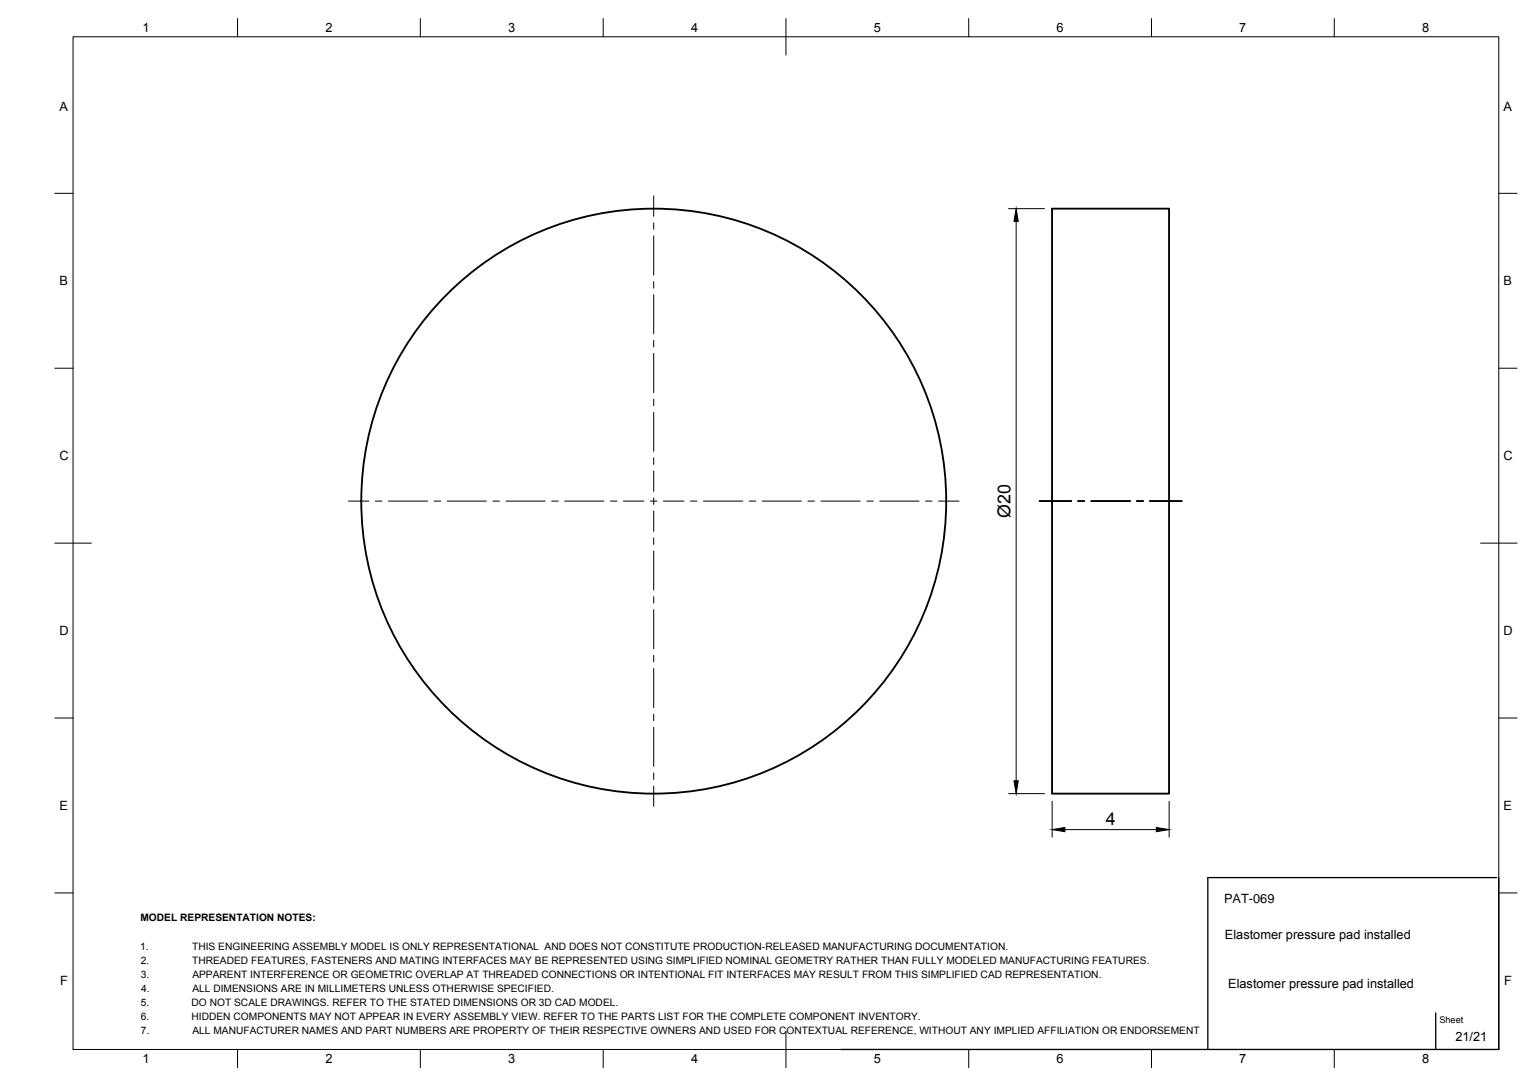
ISO-10303-21;
HEADER;
/* Generated by software containing ST-Developer
 * from STEP Tools, Inc. (www.steptools.com) 
 */

FILE_DESCRIPTION(
/* description */ ('Located fixture plate with toggle clamp'),
/* implementation_level */ '2;1');

FILE_NAME(
/* name */ 'Elastomer pressure pad installed.step',
/* time_stamp */ '2026-10-27T21:36:12-07:00',
/* author */ (''),
/* organization */ (''),
/* preprocessor_version */ 'ST-DEVELOPER v20.2',
/* originating_system */ 'Autodesk Translation Framework v15.17.0.0',
/* authorisation */ '');

FILE_SCHEMA (('AUTOMOTIVE_DESIGN { 1 0 10303 214 3 1 1 }'));
ENDSEC;

DATA;
#10=MECHANICAL_DESIGN_GEOMETRIC_PRESENTATION_REPRESENTATION('',(#340),#9285);
#292=SHAPE_REPRESENTATION_RELATIONSHIP('SRR','None',#9418,#316);
#316=ADVANCED_BREP_SHAPE_REPRESENTATION('',(#361),#9280);
#340=STYLED_ITEM('',(#9626),#361);
#361=MANIFOLD_SOLID_BREP('Body1',#5191);
#661=PLANE('',#5938);
#662=PLANE('',#5939);
#944=FACE_OUTER_BOUND('',#1352,.T.);
#945=FACE_OUTER_BOUND('',#1353,.T.);
#946=FACE_OUTER_BOUND('',#1354,.T.);
#1352=EDGE_LOOP('',(#4706,#4707,#4708,#4709));
#1353=EDGE_LOOP('',(#4710));
#1354=EDGE_LOOP('',(#4711));
#1560=CIRCLE('',#5936,1.);
#1561=CIRCLE('',#5937,1.);
#1975=LINE('',#8968,#2385);
#2385=VECTOR('',#7375,1.);
#2802=VERTEX_POINT('',#8965);
#2803=VERTEX_POINT('',#8967);
#3441=EDGE_CURVE('',#2802,#2802,#1560,.T.);
#3442=EDGE_CURVE('',#2802,#2803,#1975,.T.);
#3443=EDGE_CURVE('',#2803,#2803,#1561,.T.);
#4706=ORIENTED_EDGE('',*,*,#3441,.F.);
#4707=ORIENTED_EDGE('',*,*,#3442,.T.);
#4708=ORIENTED_EDGE('',*,*,#3443,.T.);
#4709=ORIENTED_EDGE('',*,*,#3442,.F.);
#4710=ORIENTED_EDGE('',*,*,#3441,.T.);
#4711=ORIENTED_EDGE('',*,*,#3443,.F.);
#4865=CYLINDRICAL_SURFACE('',#5935,1.);
#5145=ADVANCED_FACE('',(#944),#4865,.T.);
#5146=ADVANCED_FACE('',(#945),#661,.T.);
#5147=ADVANCED_FACE('',(#946),#662,.F.);
#5191=CLOSED_SHELL('',(#5145,#5146,#5147));
#5934=AXIS2_PLACEMENT_3D('',#8963,#7369,#7370);
#5935=AXIS2_PLACEMENT_3D('',#8964,#7371,#7372);
#5936=AXIS2_PLACEMENT_3D('',#8966,#7373,#7374);
#5937=AXIS2_PLACEMENT_3D('',#8969,#7376,#7377);
#5938=AXIS2_PLACEMENT_3D('',#8970,#7378,#7379);
#5939=AXIS2_PLACEMENT_3D('',#8971,#7380,#7381);
#7369=DIRECTION('axis',(0.,0.,1.));
#7370=DIRECTION('refdir',(1.,0.,0.));
#7371=DIRECTION('center_axis',(0.,0.,1.));
#7372=DIRECTION('ref_axis',(1.,0.,0.));
#7373=DIRECTION('center_axis',(0.,0.,1.));
#7374=DIRECTION('ref_axis',(1.,0.,0.));
#7375=DIRECTION('',(0.,0.,-1.));
#7376=DIRECTION('center_axis',(0.,0.,1.));
#7377=DIRECTION('ref_axis',(1.,0.,0.));
#7378=DIRECTION('center_axis',(0.,0.,1.));
#7379=DIRECTION('ref_axis',(1.,0.,0.));
#7380=DIRECTION('center_axis',(0.,0.,1.));
#7381=DIRECTION('ref_axis',(1.,0.,0.));
#8963=CARTESIAN_POINT('',(0.,0.,0.));
#8964=CARTESIAN_POINT('Origin',(0.,0.,3.));
#8965=CARTESIAN_POINT('',(-1.,-1.22464679914735E-16,3.4));
#8966=CARTESIAN_POINT('Origin',(0.,0.,3.4));
#8967=CARTESIAN_POINT('',(-1.,-1.22464679914735E-16,3.));
#8968=CARTESIAN_POINT('',(-1.,-1.22464679914735E-16,3.));
#8969=CARTESIAN_POINT('Origin',(0.,0.,3.));
#8970=CARTESIAN_POINT('Origin',(0.,0.,3.4));
#8971=CARTESIAN_POINT('Origin',(0.,0.,3.));
#9250=UNCERTAINTY_MEASURE_WITH_UNIT(LENGTH_MEASURE(0.001),#9286,
'DISTANCE_ACCURACY_VALUE',
'Maximum model space distance between geometric entities at asserted c
onnectivities');
#9255=UNCERTAINTY_MEASURE_WITH_UNIT(LENGTH_MEASURE(0.001),#9286,
'DISTANCE_ACCURACY_VALUE',
'Maximum model space distance between geometric entities at asserted c
onnectivities');
#9280=(
GEOMETRIC_REPRESENTATION_CONTEXT(3)
GLOBAL_UNCERTAINTY_ASSIGNED_CONTEXT((#9250))
GLOBAL_UNIT_ASSIGNED_CONTEXT((#9286,#9288,#9289))
REPRESENTATION_CONTEXT('','3D')
);
#9285=(
GEOMETRIC_REPRESENTATION_CONTEXT(3)
GLOBAL_UNCERTAINTY_ASSIGNED_CONTEXT((#9255))
GLOBAL_UNIT_ASSIGNED_CONTEXT((#9286,#9288,#9289))
REPRESENTATION_CONTEXT('','3D')
);
#9286=(
LENGTH_UNIT()
NAMED_UNIT(*)
SI_UNIT(.CENTI.,.METRE.)
);
#9288=(
NAMED_UNIT(*)
PLANE_ANGLE_UNIT()
SI_UNIT($,.RADIAN.)
);
#9289=(
NAMED_UNIT(*)
SI_UNIT($,.STERADIAN.)
SOLID_ANGLE_UNIT()
);
#9314=SHAPE_DEFINITION_REPRESENTATION(#9344,#9418);
#9344=PRODUCT_DEFINITION_SHAPE('',$,#9448);
#9418=SHAPE_REPRESENTATION('',(#5934),#9280);
#9423=PRODUCT_DEFINITION_CONTEXT('part definition',#9512,'design');
#9448=PRODUCT_DEFINITION('Elastomer pressure pad installed',
'Elastomer pressure pad installed',#9477,#9423);
#9477=PRODUCT_DEFINITION_FORMATION('',$,#9538);
#9512=APPLICATION_CONTEXT(
'Core Data for Automotive Mechanical Design Process');
#9513=PRODUCT_CONTEXT('part definition',#9512,'mechanical');
#9538=PRODUCT('Elastomer pressure pad installed',
'Elastomer pressure pad installed','Elastomer pressure pad installed',(#9513));
#9620=COLOUR_RGB('Off White',0.89,0.88,0.83);
#9621=FILL_AREA_STYLE_COLOUR('',#9620);
#9622=FILL_AREA_STYLE('',(#9621));
#9623=SURFACE_STYLE_FILL_AREA(#9622);
#9624=SURFACE_SIDE_STYLE('',(#9623));
#9625=SURFACE_STYLE_USAGE(.BOTH.,#9624);
#9626=PRESENTATION_STYLE_ASSIGNMENT((#9625));
ENDSEC;
END-ISO-10303-21;
